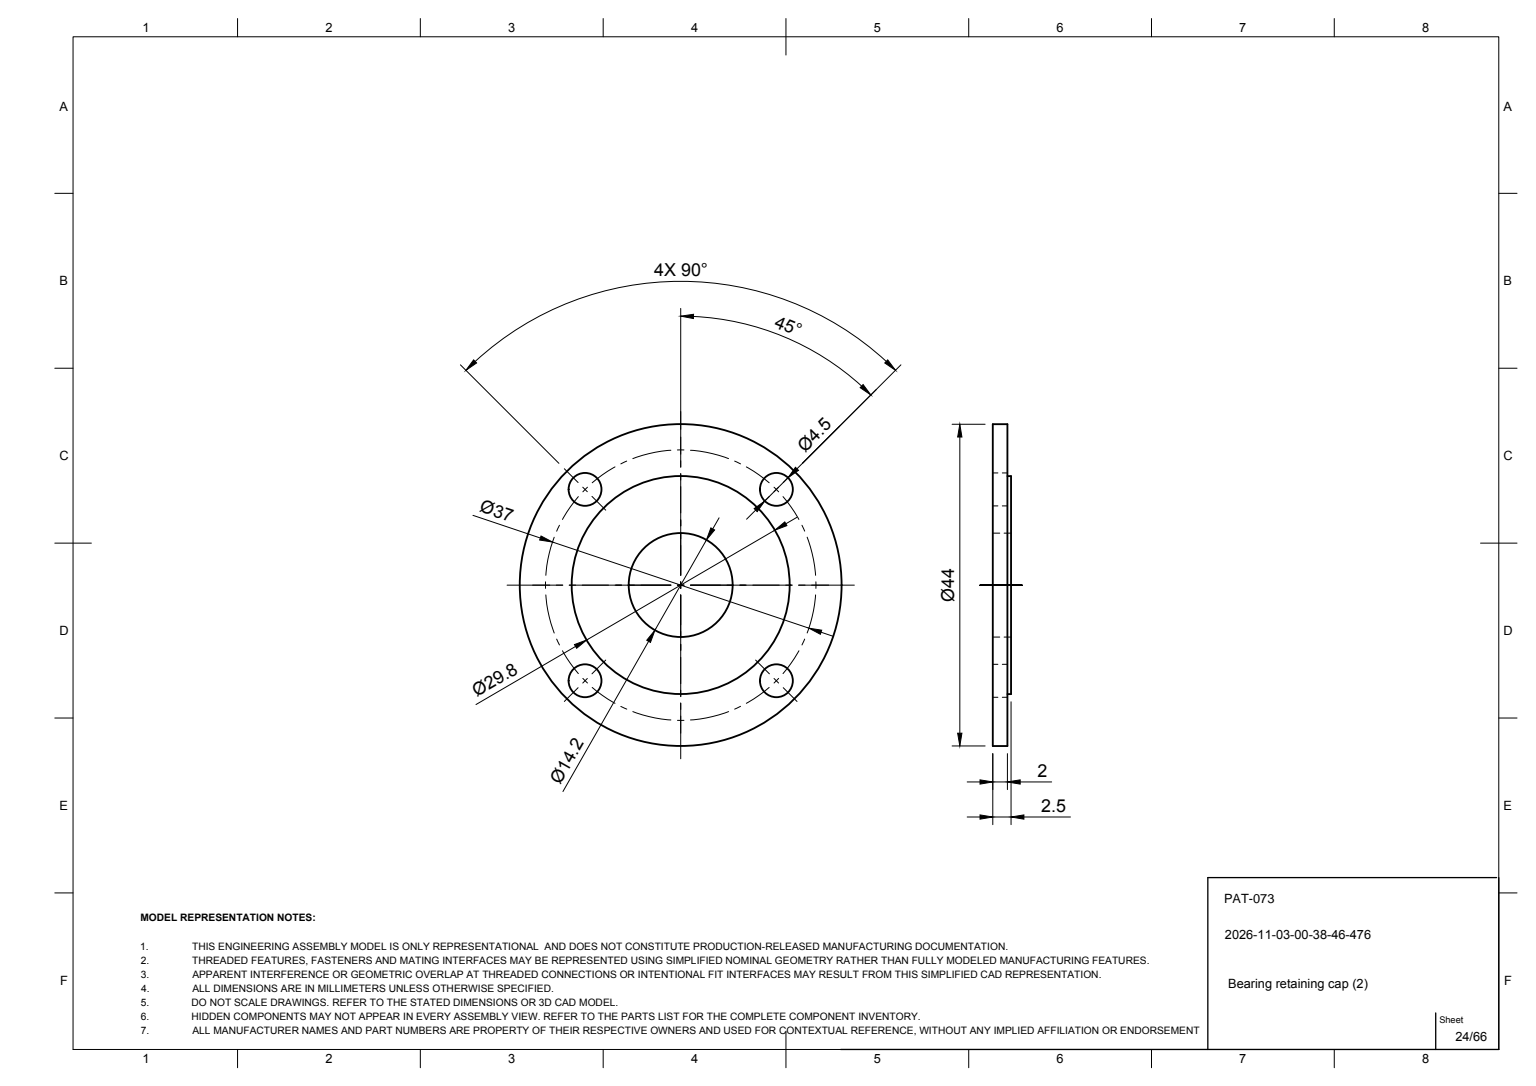
ISO-10303-21;
HEADER;
/* Generated by software containing ST-Developer
 * from STEP Tools, Inc. (www.steptools.com) 
 */

FILE_DESCRIPTION(
/* description */ ('Manual piston pump'),
/* implementation_level */ '2;1');

FILE_NAME(
/* name */ 'Bearing retaining cap (2).step',
/* time_stamp */ '2026-11-02T16:54:23-08:00',
/* author */ (''),
/* organization */ (''),
/* preprocessor_version */ 'ST-DEVELOPER v20.2',
/* originating_system */ 'Autodesk Translation Framework v15.17.0.0',
/* authorisation */ '');

FILE_SCHEMA (('AUTOMOTIVE_DESIGN { 1 0 10303 214 3 1 1 }'));
ENDSEC;

DATA;
#10=MECHANICAL_DESIGN_GEOMETRIC_PRESENTATION_REPRESENTATION('',(#724),#19043);
#590=SHAPE_REPRESENTATION_RELATIONSHIP('SRR','None',#19337,#653);
#653=ADVANCED_BREP_SHAPE_REPRESENTATION('',(#794),#19004);
#724=STYLED_ITEM('',(#19664),#794);
#794=MANIFOLD_SOLID_BREP('Body1',#9510);
#955=FACE_BOUND('',#2290,.T.);
#956=FACE_BOUND('',#2294,.T.);
#957=FACE_BOUND('',#2295,.T.);
#958=FACE_BOUND('',#2296,.T.);
#959=FACE_BOUND('',#2297,.T.);
#960=FACE_BOUND('',#2298,.T.);
#961=FACE_BOUND('',#2300,.T.);
#962=FACE_BOUND('',#2301,.T.);
#963=FACE_BOUND('',#2302,.T.);
#964=FACE_BOUND('',#2303,.T.);
#965=FACE_BOUND('',#2304,.T.);
#1195=CYLINDRICAL_SURFACE('',#10839,0.225);
#1196=CYLINDRICAL_SURFACE('',#10842,0.225);
#1197=CYLINDRICAL_SURFACE('',#10845,0.225);
#1198=CYLINDRICAL_SURFACE('',#10848,0.225);
#1199=CYLINDRICAL_SURFACE('',#10851,1.49);
#1200=CYLINDRICAL_SURFACE('',#10856,0.710000000000001);
#1201=CYLINDRICAL_SURFACE('',#10858,2.2);
#1581=FACE_OUTER_BOUND('',#2284,.T.);
#1582=FACE_OUTER_BOUND('',#2285,.T.);
#1583=FACE_OUTER_BOUND('',#2286,.T.);
#1584=FACE_OUTER_BOUND('',#2287,.T.);
#1585=FACE_OUTER_BOUND('',#2288,.T.);
#1586=FACE_OUTER_BOUND('',#2289,.T.);
#1587=FACE_OUTER_BOUND('',#2291,.T.);
#1588=FACE_OUTER_BOUND('',#2292,.T.);
#1589=FACE_OUTER_BOUND('',#2293,.T.);
#1590=FACE_OUTER_BOUND('',#2299,.T.);
#2284=EDGE_LOOP('',(#7461,#7462,#7463,#7464));
#2285=EDGE_LOOP('',(#7465,#7466,#7467,#7468));
#2286=EDGE_LOOP('',(#7469,#7470,#7471,#7472));
#2287=EDGE_LOOP('',(#7473,#7474,#7475,#7476));
#2288=EDGE_LOOP('',(#7477,#7478,#7479,#7480));
#2289=EDGE_LOOP('',(#7481));
#2290=EDGE_LOOP('',(#7482));
#2291=EDGE_LOOP('',(#7483,#7484,#7485,#7486));
#2292=EDGE_LOOP('',(#7487,#7488,#7489,#7490));
#2293=EDGE_LOOP('',(#7491));
#2294=EDGE_LOOP('',(#7492));
#2295=EDGE_LOOP('',(#7493));
#2296=EDGE_LOOP('',(#7494));
#2297=EDGE_LOOP('',(#7495));
#2298=EDGE_LOOP('',(#7496));
#2299=EDGE_LOOP('',(#7497));
#2300=EDGE_LOOP('',(#7498));
#2301=EDGE_LOOP('',(#7499));
#2302=EDGE_LOOP('',(#7500));
#2303=EDGE_LOOP('',(#7501));
#2304=EDGE_LOOP('',(#7502));
#2933=CIRCLE('',#10840,0.225);
#2934=CIRCLE('',#10841,0.225);
#2935=CIRCLE('',#10843,0.225);
#2936=CIRCLE('',#10844,0.225);
#2937=CIRCLE('',#10846,0.225);
#2938=CIRCLE('',#10847,0.225);
#2939=CIRCLE('',#10849,0.225);
#2940=CIRCLE('',#10850,0.225);
#2941=CIRCLE('',#10852,1.49);
#2942=CIRCLE('',#10853,1.49);
#2943=CIRCLE('',#10855,0.710000000000001);
#2944=CIRCLE('',#10857,0.710000000000001);
#2945=CIRCLE('',#10859,2.2);
#2946=CIRCLE('',#10860,2.2);
#3438=LINE('',#16341,#4042);
#3439=LINE('',#16347,#4043);
#3440=LINE('',#16353,#4044);
#3441=LINE('',#16359,#4045);
#3442=LINE('',#16365,#4046);
#3443=LINE('',#16372,#4047);
#3444=LINE('',#16378,#4048);
#4042=VECTOR('',#12982,0.225);
#4043=VECTOR('',#12989,0.225);
#4044=VECTOR('',#12996,0.225);
#4045=VECTOR('',#13003,0.225);
#4046=VECTOR('',#13010,1.49);
#4047=VECTOR('',#13019,0.710000000000001);
#4048=VECTOR('',#13026,2.2);
#4756=VERTEX_POINT('',#16338);
#4757=VERTEX_POINT('',#16340);
#4758=VERTEX_POINT('',#16344);
#4759=VERTEX_POINT('',#16346);
#4760=VERTEX_POINT('',#16350);
#4761=VERTEX_POINT('',#16352);
#4762=VERTEX_POINT('',#16356);
#4763=VERTEX_POINT('',#16358);
#4764=VERTEX_POINT('',#16362);
#4765=VERTEX_POINT('',#16364);
#4766=VERTEX_POINT('',#16368);
#4767=VERTEX_POINT('',#16371);
#4768=VERTEX_POINT('',#16375);
#4769=VERTEX_POINT('',#16377);
#5717=EDGE_CURVE('',#4756,#4756,#2933,.T.);
#5718=EDGE_CURVE('',#4756,#4757,#3438,.T.);
#5719=EDGE_CURVE('',#4757,#4757,#2934,.T.);
#5720=EDGE_CURVE('',#4758,#4758,#2935,.T.);
#5721=EDGE_CURVE('',#4758,#4759,#3439,.T.);
#5722=EDGE_CURVE('',#4759,#4759,#2936,.T.);
#5723=EDGE_CURVE('',#4760,#4760,#2937,.T.);
#5724=EDGE_CURVE('',#4760,#4761,#3440,.T.);
#5725=EDGE_CURVE('',#4761,#4761,#2938,.T.);
#5726=EDGE_CURVE('',#4762,#4762,#2939,.T.);
#5727=EDGE_CURVE('',#4762,#4763,#3441,.T.);
#5728=EDGE_CURVE('',#4763,#4763,#2940,.T.);
#5729=EDGE_CURVE('',#4764,#4764,#2941,.T.);
#5730=EDGE_CURVE('',#4764,#4765,#3442,.T.);
#5731=EDGE_CURVE('',#4765,#4765,#2942,.T.);
#5732=EDGE_CURVE('',#4766,#4766,#2943,.T.);
#5733=EDGE_CURVE('',#4766,#4767,#3443,.T.);
#5734=EDGE_CURVE('',#4767,#4767,#2944,.T.);
#5735=EDGE_CURVE('',#4768,#4768,#2945,.T.);
#5736=EDGE_CURVE('',#4768,#4769,#3444,.T.);
#5737=EDGE_CURVE('',#4769,#4769,#2946,.T.);
#7461=ORIENTED_EDGE('',*,*,#5717,.F.);
#7462=ORIENTED_EDGE('',*,*,#5718,.T.);
#7463=ORIENTED_EDGE('',*,*,#5719,.F.);
#7464=ORIENTED_EDGE('',*,*,#5718,.F.);
#7465=ORIENTED_EDGE('',*,*,#5720,.F.);
#7466=ORIENTED_EDGE('',*,*,#5721,.T.);
#7467=ORIENTED_EDGE('',*,*,#5722,.F.);
#7468=ORIENTED_EDGE('',*,*,#5721,.F.);
#7469=ORIENTED_EDGE('',*,*,#5723,.F.);
#7470=ORIENTED_EDGE('',*,*,#5724,.T.);
#7471=ORIENTED_EDGE('',*,*,#5725,.F.);
#7472=ORIENTED_EDGE('',*,*,#5724,.F.);
#7473=ORIENTED_EDGE('',*,*,#5726,.F.);
#7474=ORIENTED_EDGE('',*,*,#5727,.T.);
#7475=ORIENTED_EDGE('',*,*,#5728,.F.);
#7476=ORIENTED_EDGE('',*,*,#5727,.F.);
#7477=ORIENTED_EDGE('',*,*,#5729,.F.);
#7478=ORIENTED_EDGE('',*,*,#5730,.T.);
#7479=ORIENTED_EDGE('',*,*,#5731,.F.);
#7480=ORIENTED_EDGE('',*,*,#5730,.F.);
#7481=ORIENTED_EDGE('',*,*,#5729,.T.);
#7482=ORIENTED_EDGE('',*,*,#5732,.T.);
#7483=ORIENTED_EDGE('',*,*,#5732,.F.);
#7484=ORIENTED_EDGE('',*,*,#5733,.T.);
#7485=ORIENTED_EDGE('',*,*,#5734,.T.);
#7486=ORIENTED_EDGE('',*,*,#5733,.F.);
#7487=ORIENTED_EDGE('',*,*,#5735,.F.);
#7488=ORIENTED_EDGE('',*,*,#5736,.T.);
#7489=ORIENTED_EDGE('',*,*,#5737,.T.);
#7490=ORIENTED_EDGE('',*,*,#5736,.F.);
#7491=ORIENTED_EDGE('',*,*,#5735,.T.);
#7492=ORIENTED_EDGE('',*,*,#5731,.T.);
#7493=ORIENTED_EDGE('',*,*,#5728,.T.);
#7494=ORIENTED_EDGE('',*,*,#5725,.T.);
#7495=ORIENTED_EDGE('',*,*,#5722,.T.);
#7496=ORIENTED_EDGE('',*,*,#5719,.T.);
#7497=ORIENTED_EDGE('',*,*,#5737,.F.);
#7498=ORIENTED_EDGE('',*,*,#5734,.F.);
#7499=ORIENTED_EDGE('',*,*,#5726,.T.);
#7500=ORIENTED_EDGE('',*,*,#5723,.T.);
#7501=ORIENTED_EDGE('',*,*,#5720,.T.);
#7502=ORIENTED_EDGE('',*,*,#5717,.T.);
#8725=PLANE('',#10854);
#8726=PLANE('',#10861);
#8727=PLANE('',#10862);
#9186=ADVANCED_FACE('',(#1581),#1195,.F.);
#9187=ADVANCED_FACE('',(#1582),#1196,.F.);
#9188=ADVANCED_FACE('',(#1583),#1197,.F.);
#9189=ADVANCED_FACE('',(#1584),#1198,.F.);
#9190=ADVANCED_FACE('',(#1585),#1199,.T.);
#9191=ADVANCED_FACE('',(#1586,#955),#8725,.T.);
#9192=ADVANCED_FACE('',(#1587),#1200,.F.);
#9193=ADVANCED_FACE('',(#1588),#1201,.T.);
#9194=ADVANCED_FACE('',(#1589,#956,#957,#958,#959,#960),#8726,.T.);
#9195=ADVANCED_FACE('',(#1590,#961,#962,#963,#964,#965),#8727,.F.);
#9510=CLOSED_SHELL('',(#9186,#9187,#9188,#9189,#9190,#9191,#9192,#9193,
#9194,#9195));
#10838=AXIS2_PLACEMENT_3D('',#16336,#12976,#12977);
#10839=AXIS2_PLACEMENT_3D('',#16337,#12978,#12979);
#10840=AXIS2_PLACEMENT_3D('',#16339,#12980,#12981);
#10841=AXIS2_PLACEMENT_3D('',#16342,#12983,#12984);
#10842=AXIS2_PLACEMENT_3D('',#16343,#12985,#12986);
#10843=AXIS2_PLACEMENT_3D('',#16345,#12987,#12988);
#10844=AXIS2_PLACEMENT_3D('',#16348,#12990,#12991);
#10845=AXIS2_PLACEMENT_3D('',#16349,#12992,#12993);
#10846=AXIS2_PLACEMENT_3D('',#16351,#12994,#12995);
#10847=AXIS2_PLACEMENT_3D('',#16354,#12997,#12998);
#10848=AXIS2_PLACEMENT_3D('',#16355,#12999,#13000);
#10849=AXIS2_PLACEMENT_3D('',#16357,#13001,#13002);
#10850=AXIS2_PLACEMENT_3D('',#16360,#13004,#13005);
#10851=AXIS2_PLACEMENT_3D('',#16361,#13006,#13007);
#10852=AXIS2_PLACEMENT_3D('',#16363,#13008,#13009);
#10853=AXIS2_PLACEMENT_3D('',#16366,#13011,#13012);
#10854=AXIS2_PLACEMENT_3D('',#16367,#13013,#13014);
#10855=AXIS2_PLACEMENT_3D('',#16369,#13015,#13016);
#10856=AXIS2_PLACEMENT_3D('',#16370,#13017,#13018);
#10857=AXIS2_PLACEMENT_3D('',#16373,#13020,#13021);
#10858=AXIS2_PLACEMENT_3D('',#16374,#13022,#13023);
#10859=AXIS2_PLACEMENT_3D('',#16376,#13024,#13025);
#10860=AXIS2_PLACEMENT_3D('',#16379,#13027,#13028);
#10861=AXIS2_PLACEMENT_3D('',#16380,#13029,#13030);
#10862=AXIS2_PLACEMENT_3D('',#16381,#13031,#13032);
#12976=DIRECTION('axis',(0.,0.,1.));
#12977=DIRECTION('refdir',(1.,0.,0.));
#12978=DIRECTION('center_axis',(1.,0.,0.));
#12979=DIRECTION('ref_axis',(0.,0.,-1.));
#12980=DIRECTION('center_axis',(1.,0.,0.));
#12981=DIRECTION('ref_axis',(0.,0.,-1.));
#12982=DIRECTION('',(1.,0.,0.));
#12983=DIRECTION('center_axis',(-1.,0.,0.));
#12984=DIRECTION('ref_axis',(0.,0.,-1.));
#12985=DIRECTION('center_axis',(1.,0.,0.));
#12986=DIRECTION('ref_axis',(0.,0.,-1.));
#12987=DIRECTION('center_axis',(1.,0.,0.));
#12988=DIRECTION('ref_axis',(0.,0.,-1.));
#12989=DIRECTION('',(1.,0.,0.));
#12990=DIRECTION('center_axis',(-1.,0.,0.));
#12991=DIRECTION('ref_axis',(0.,0.,-1.));
#12992=DIRECTION('center_axis',(1.,0.,0.));
#12993=DIRECTION('ref_axis',(0.,0.,-1.));
#12994=DIRECTION('center_axis',(1.,0.,0.));
#12995=DIRECTION('ref_axis',(0.,0.,-1.));
#12996=DIRECTION('',(1.,0.,0.));
#12997=DIRECTION('center_axis',(-1.,0.,0.));
#12998=DIRECTION('ref_axis',(0.,0.,-1.));
#12999=DIRECTION('center_axis',(1.,0.,0.));
#13000=DIRECTION('ref_axis',(0.,0.,-1.));
#13001=DIRECTION('center_axis',(1.,0.,0.));
#13002=DIRECTION('ref_axis',(0.,0.,-1.));
#13003=DIRECTION('',(1.,0.,0.));
#13004=DIRECTION('center_axis',(-1.,0.,0.));
#13005=DIRECTION('ref_axis',(0.,0.,-1.));
#13006=DIRECTION('center_axis',(1.,0.,0.));
#13007=DIRECTION('ref_axis',(0.,0.,-1.));
#13008=DIRECTION('center_axis',(1.,0.,0.));
#13009=DIRECTION('ref_axis',(0.,0.,-1.));
#13010=DIRECTION('',(-1.,0.,0.));
#13011=DIRECTION('center_axis',(-1.,0.,0.));
#13012=DIRECTION('ref_axis',(0.,0.,-1.));
#13013=DIRECTION('center_axis',(1.,0.,0.));
#13014=DIRECTION('ref_axis',(0.,0.,-1.));
#13015=DIRECTION('center_axis',(-1.,0.,0.));
#13016=DIRECTION('ref_axis',(0.,0.,-1.));
#13017=DIRECTION('center_axis',(1.,0.,0.));
#13018=DIRECTION('ref_axis',(0.,0.,-1.));
#13019=DIRECTION('',(-1.,0.,0.));
#13020=DIRECTION('center_axis',(-1.,0.,0.));
#13021=DIRECTION('ref_axis',(0.,0.,-1.));
#13022=DIRECTION('center_axis',(1.,0.,0.));
#13023=DIRECTION('ref_axis',(0.,0.,-1.));
#13024=DIRECTION('center_axis',(1.,0.,0.));
#13025=DIRECTION('ref_axis',(0.,0.,-1.));
#13026=DIRECTION('',(-1.,0.,0.));
#13027=DIRECTION('center_axis',(1.,0.,0.));
#13028=DIRECTION('ref_axis',(0.,0.,-1.));
#13029=DIRECTION('center_axis',(1.,0.,0.));
#13030=DIRECTION('ref_axis',(0.,0.,-1.));
#13031=DIRECTION('center_axis',(1.,0.,0.));
#13032=DIRECTION('ref_axis',(0.,0.,-1.));
#16336=CARTESIAN_POINT('',(0.,0.,0.));
#16337=CARTESIAN_POINT('Origin',(2.7,-5.30814754519511,8.69185245480489));
#16338=CARTESIAN_POINT('',(2.8,-5.30814754519511,8.91685245480489));
#16339=CARTESIAN_POINT('Origin',(2.8,-5.30814754519511,8.69185245480489));
#16340=CARTESIAN_POINT('',(3.,-5.30814754519511,8.91685245480489));
#16341=CARTESIAN_POINT('',(2.7,-5.30814754519511,8.91685245480489));
#16342=CARTESIAN_POINT('Origin',(3.,-5.30814754519511,8.69185245480489));
#16343=CARTESIAN_POINT('Origin',(2.7,-5.30814754519511,11.3081475451951));
#16344=CARTESIAN_POINT('',(2.8,-5.30814754519511,11.5331475451951));
#16345=CARTESIAN_POINT('Origin',(2.8,-5.30814754519511,11.3081475451951));
#16346=CARTESIAN_POINT('',(3.,-5.30814754519511,11.5331475451951));
#16347=CARTESIAN_POINT('',(2.7,-5.30814754519511,11.5331475451951));
#16348=CARTESIAN_POINT('Origin',(3.,-5.30814754519511,11.3081475451951));
#16349=CARTESIAN_POINT('Origin',(2.7,-2.69185245480489,11.3081475451951));
#16350=CARTESIAN_POINT('',(2.8,-2.69185245480489,11.5331475451951));
#16351=CARTESIAN_POINT('Origin',(2.8,-2.69185245480489,11.3081475451951));
#16352=CARTESIAN_POINT('',(3.,-2.69185245480489,11.5331475451951));
#16353=CARTESIAN_POINT('',(2.7,-2.69185245480489,11.5331475451951));
#16354=CARTESIAN_POINT('Origin',(3.,-2.69185245480489,11.3081475451951));
#16355=CARTESIAN_POINT('Origin',(2.7,-2.69185245480489,8.69185245480489));
#16356=CARTESIAN_POINT('',(2.8,-2.69185245480489,8.91685245480489));
#16357=CARTESIAN_POINT('Origin',(2.8,-2.69185245480489,8.69185245480489));
#16358=CARTESIAN_POINT('',(3.,-2.69185245480489,8.91685245480489));
#16359=CARTESIAN_POINT('',(2.7,-2.69185245480489,8.91685245480489));
#16360=CARTESIAN_POINT('Origin',(3.,-2.69185245480489,8.69185245480489));
#16361=CARTESIAN_POINT('Origin',(3.,-4.,10.));
#16362=CARTESIAN_POINT('',(3.05,-4.,11.49));
#16363=CARTESIAN_POINT('Origin',(3.05,-4.,10.));
#16364=CARTESIAN_POINT('',(3.,-4.,11.49));
#16365=CARTESIAN_POINT('',(3.,-4.,11.49));
#16366=CARTESIAN_POINT('Origin',(3.,-4.,10.));
#16367=CARTESIAN_POINT('Origin',(3.05,-4.,10.));
#16368=CARTESIAN_POINT('',(3.05,-4.,10.71));
#16369=CARTESIAN_POINT('Origin',(3.05,-4.,10.));
#16370=CARTESIAN_POINT('Origin',(2.8,-4.,10.));
#16371=CARTESIAN_POINT('',(2.8,-4.,10.71));
#16372=CARTESIAN_POINT('',(2.8,-4.,10.71));
#16373=CARTESIAN_POINT('Origin',(2.8,-4.,10.));
#16374=CARTESIAN_POINT('Origin',(2.8,-4.,10.));
#16375=CARTESIAN_POINT('',(3.,-4.,12.2));
#16376=CARTESIAN_POINT('Origin',(3.,-4.,10.));
#16377=CARTESIAN_POINT('',(2.8,-4.,12.2));
#16378=CARTESIAN_POINT('',(2.8,-4.,12.2));
#16379=CARTESIAN_POINT('Origin',(2.8,-4.,10.));
#16380=CARTESIAN_POINT('Origin',(3.,-4.,10.));
#16381=CARTESIAN_POINT('Origin',(2.8,-4.,10.));
#18933=UNCERTAINTY_MEASURE_WITH_UNIT(LENGTH_MEASURE(0.001),#19044,
'DISTANCE_ACCURACY_VALUE',
'Maximum model space distance between geometric entities at asserted c
onnectivities');
#18972=UNCERTAINTY_MEASURE_WITH_UNIT(LENGTH_MEASURE(0.001),#19044,
'DISTANCE_ACCURACY_VALUE',
'Maximum model space distance between geometric entities at asserted c
onnectivities');
#19004=(
GEOMETRIC_REPRESENTATION_CONTEXT(3)
GLOBAL_UNCERTAINTY_ASSIGNED_CONTEXT((#18933))
GLOBAL_UNIT_ASSIGNED_CONTEXT((#19044,#19046,#19047))
REPRESENTATION_CONTEXT('','3D')
);
#19043=(
GEOMETRIC_REPRESENTATION_CONTEXT(3)
GLOBAL_UNCERTAINTY_ASSIGNED_CONTEXT((#18972))
GLOBAL_UNIT_ASSIGNED_CONTEXT((#19044,#19046,#19047))
REPRESENTATION_CONTEXT('','3D')
);
#19044=(
LENGTH_UNIT()
NAMED_UNIT(*)
SI_UNIT(.CENTI.,.METRE.)
);
#19046=(
NAMED_UNIT(*)
PLANE_ANGLE_UNIT()
SI_UNIT($,.RADIAN.)
);
#19047=(
NAMED_UNIT(*)
SI_UNIT($,.STERADIAN.)
SOLID_ANGLE_UNIT()
);
#19079=SHAPE_DEFINITION_REPRESENTATION(#19154,#19337);
#19154=PRODUCT_DEFINITION_SHAPE('',$,#19408);
#19337=SHAPE_REPRESENTATION('',(#10838),#19004);
#19376=PRODUCT_DEFINITION_CONTEXT('part definition',#19588,'design');
#19408=PRODUCT_DEFINITION('2026-11-03-00-38-46-476',
'Bearing retaining cap (2)',#19478,#19376);
#19478=PRODUCT_DEFINITION_FORMATION('',$,#19621);
#19588=APPLICATION_CONTEXT(
'Core Data for Automotive Mechanical Design Process');
#19589=PRODUCT_CONTEXT('part definition',#19588,'mechanical');
#19621=PRODUCT('2026-11-03-00-38-46-476','Bearing retaining cap (2)',
'Bearing retaining cap',(#19589));
#19664=PRESENTATION_STYLE_ASSIGNMENT((#19670));
#19670=SURFACE_STYLE_USAGE(.BOTH.,#19676);
#19676=SURFACE_SIDE_STYLE('',(#19682));
#19682=SURFACE_STYLE_FILL_AREA(#19688);
#19688=FILL_AREA_STYLE('CAD Library Painted - Steel gray',(#19694));
#19694=FILL_AREA_STYLE_COLOUR('CAD Library Painted - Steel gray',#19700);
#19700=COLOUR_RGB('CAD Library Painted - Steel gray',0.592156862745098,
0.631372549019608,0.67843137254902);
ENDSEC;
END-ISO-10303-21;
